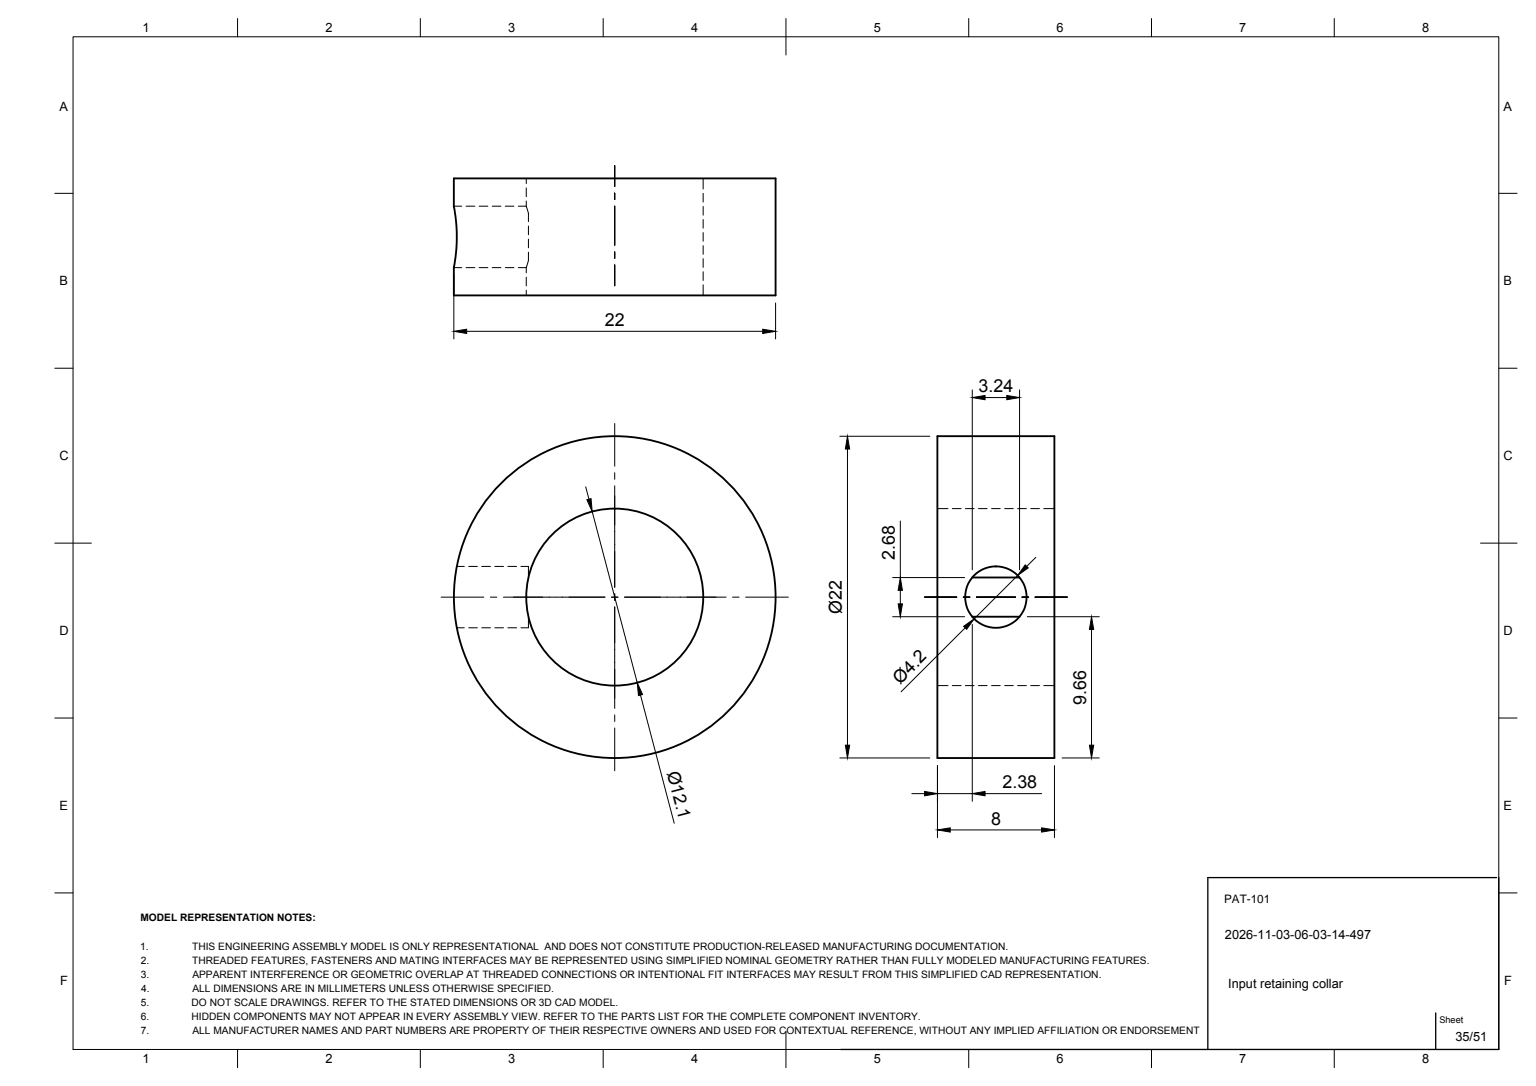
ISO-10303-21;
HEADER;
/* Generated by software containing ST-Developer
 * from STEP Tools, Inc. (www.steptools.com) 
 */

FILE_DESCRIPTION(
/* description */ ('Spur gear reduction stage 2-1 on bearing plates'),
/* implementation_level */ '2;1');

FILE_NAME(
/* name */ 'Input retaining collar.step',
/* time_stamp */ '2026-10-28T03:22:07-07:00',
/* author */ (''),
/* organization */ (''),
/* preprocessor_version */ 'ST-DEVELOPER v20.2',
/* originating_system */ 'Autodesk Translation Framework v15.17.0.0',
/* authorisation */ '');

FILE_SCHEMA (('AUTOMOTIVE_DESIGN { 1 0 10303 214 3 1 1 }'));
ENDSEC;

DATA;
#10=MECHANICAL_DESIGN_GEOMETRIC_PRESENTATION_REPRESENTATION('',(#989),#53909);
#699=B_SPLINE_CURVE_WITH_KNOTS('',3,(#17992,#17993,#17994,#17995,#17996,
#17997,#17998,#17999,#18000,#18001),.UNSPECIFIED.,.F.,.F.,(4,2,2,2,4),(0.818088904349169,
0.878131747417165,0.957937926194036,1.03774410497091,1.0977869480389),
 .UNSPECIFIED.);
#700=B_SPLINE_CURVE_WITH_KNOTS('',3,(#18007,#18008,#18009,#18010,#18011,
#18012,#18013,#18014,#18015,#18016,#18017,#18018,#18019,#18020,#18021,#18022,
#18023,#18024),.UNSPECIFIED.,.F.,.F.,(4,2,2,2,2,2,2,2,4),(0.,0.0793157643915219,
0.158631528783044,0.23794361593365,0.317255703084255,0.396567790234861,
0.475879877385467,0.555195641776989,0.634511406168511),.UNSPECIFIED.);
#701=B_SPLINE_CURVE_WITH_KNOTS('',3,(#18025,#18026,#18027,#18028,#18029,
#18030,#18031,#18032,#18033,#18034,#18035,#18036,#18037,#18038,#18039,#18040,
#18041,#18042),.UNSPECIFIED.,.F.,.F.,(4,2,2,2,2,2,2,2,4),(0.634511406168511,
0.713827170560033,0.793142934951554,0.87245502210216,0.951767109252766,
1.03107919640337,1.11039128355398,1.1897070479455,1.26902281233702),
 .UNSPECIFIED.);
#702=B_SPLINE_CURVE_WITH_KNOTS('',3,(#18045,#18046,#18047,#18048,#18049,
#18050,#18051,#18052,#18053,#18054),.UNSPECIFIED.,.F.,.F.,(4,2,2,2,4),(0.179463620219812,
0.239506463287808,0.319312642064679,0.399118820841549,0.459161663909545),
 .UNSPECIFIED.);
#888=SHAPE_REPRESENTATION_RELATIONSHIP('SRR','None',#54118,#931);
#931=ADVANCED_BREP_SHAPE_REPRESENTATION('',(#1044),#53892);
#989=STYLED_ITEM('',(#54383),#1044);
#1044=MANIFOLD_SOLID_BREP('Body1',#11316);
#1202=FACE_BOUND('',#2593,.T.);
#1203=FACE_BOUND('',#2595,.T.);
#1204=FACE_BOUND('',#2597,.T.);
#1205=FACE_BOUND('',#2599,.T.);
#1369=PLANE('',#12513);
#1370=PLANE('',#12518);
#1371=PLANE('',#12525);
#1372=PLANE('',#12526);
#1799=FACE_OUTER_BOUND('',#2589,.T.);
#1800=FACE_OUTER_BOUND('',#2590,.T.);
#1801=FACE_OUTER_BOUND('',#2591,.T.);
#1802=FACE_OUTER_BOUND('',#2592,.T.);
#1803=FACE_OUTER_BOUND('',#2594,.T.);
#1804=FACE_OUTER_BOUND('',#2596,.T.);
#1805=FACE_OUTER_BOUND('',#2598,.T.);
#2589=EDGE_LOOP('',(#8536,#8537));
#2590=EDGE_LOOP('',(#8538,#8539,#8540,#8541,#8542,#8543,#8544,#8545,#8546));
#2591=EDGE_LOOP('',(#8547,#8548,#8549));
#2592=EDGE_LOOP('',(#8550,#8551,#8552,#8553));
#2593=EDGE_LOOP('',(#8554,#8555,#8556,#8557));
#2594=EDGE_LOOP('',(#8558,#8559,#8560,#8561));
#2595=EDGE_LOOP('',(#8562,#8563));
#2596=EDGE_LOOP('',(#8564));
#2597=EDGE_LOOP('',(#8565));
#2598=EDGE_LOOP('',(#8566));
#2599=EDGE_LOOP('',(#8567));
#3208=LINE('',#17988,#3849);
#3209=LINE('',#18005,#3850);
#3210=LINE('',#18056,#3851);
#3211=LINE('',#18061,#3852);
#3212=LINE('',#18067,#3853);
#3849=VECTOR('',#14629,1.);
#3850=VECTOR('',#14636,0.21);
#3851=VECTOR('',#14641,1.);
#3852=VECTOR('',#14646,0.605);
#3853=VECTOR('',#14653,1.1);
#4588=CIRCLE('',#12514,0.21);
#4589=CIRCLE('',#12516,0.21);
#4590=CIRCLE('',#12517,0.21);
#4591=CIRCLE('',#12520,0.605);
#4592=CIRCLE('',#12521,0.605);
#4593=CIRCLE('',#12523,1.1);
#4594=CIRCLE('',#12524,1.1);
#5192=VERTEX_POINT('',#17986);
#5193=VERTEX_POINT('',#17987);
#5194=VERTEX_POINT('',#17991);
#5195=VERTEX_POINT('',#18002);
#5196=VERTEX_POINT('',#18004);
#5197=VERTEX_POINT('',#18006);
#5198=VERTEX_POINT('',#18043);
#5199=VERTEX_POINT('',#18058);
#5200=VERTEX_POINT('',#18060);
#5201=VERTEX_POINT('',#18064);
#5202=VERTEX_POINT('',#18066);
#6410=EDGE_CURVE('',#5192,#5193,#3208,.T.);
#6411=EDGE_CURVE('',#5192,#5193,#4588,.T.);
#6412=EDGE_CURVE('',#5194,#5192,#699,.T.);
#6413=EDGE_CURVE('',#5195,#5194,#4589,.T.);
#6414=EDGE_CURVE('',#5195,#5196,#3209,.T.);
#6415=EDGE_CURVE('',#5197,#5196,#700,.T.);
#6416=EDGE_CURVE('',#5196,#5197,#701,.T.);
#6417=EDGE_CURVE('',#5198,#5195,#4590,.T.);
#6418=EDGE_CURVE('',#5193,#5198,#702,.T.);
#6419=EDGE_CURVE('',#5198,#5194,#3210,.T.);
#6420=EDGE_CURVE('',#5199,#5199,#4591,.T.);
#6421=EDGE_CURVE('',#5199,#5200,#3211,.T.);
#6422=EDGE_CURVE('',#5200,#5200,#4592,.T.);
#6423=EDGE_CURVE('',#5201,#5201,#4593,.T.);
#6424=EDGE_CURVE('',#5201,#5202,#3212,.T.);
#6425=EDGE_CURVE('',#5202,#5202,#4594,.T.);
#8536=ORIENTED_EDGE('',*,*,#6410,.F.);
#8537=ORIENTED_EDGE('',*,*,#6411,.T.);
#8538=ORIENTED_EDGE('',*,*,#6412,.F.);
#8539=ORIENTED_EDGE('',*,*,#6413,.F.);
#8540=ORIENTED_EDGE('',*,*,#6414,.T.);
#8541=ORIENTED_EDGE('',*,*,#6415,.F.);
#8542=ORIENTED_EDGE('',*,*,#6416,.F.);
#8543=ORIENTED_EDGE('',*,*,#6414,.F.);
#8544=ORIENTED_EDGE('',*,*,#6417,.F.);
#8545=ORIENTED_EDGE('',*,*,#6418,.F.);
#8546=ORIENTED_EDGE('',*,*,#6411,.F.);
#8547=ORIENTED_EDGE('',*,*,#6419,.F.);
#8548=ORIENTED_EDGE('',*,*,#6417,.T.);
#8549=ORIENTED_EDGE('',*,*,#6413,.T.);
#8550=ORIENTED_EDGE('',*,*,#6420,.F.);
#8551=ORIENTED_EDGE('',*,*,#6421,.T.);
#8552=ORIENTED_EDGE('',*,*,#6422,.T.);
#8553=ORIENTED_EDGE('',*,*,#6421,.F.);
#8554=ORIENTED_EDGE('',*,*,#6418,.T.);
#8555=ORIENTED_EDGE('',*,*,#6419,.T.);
#8556=ORIENTED_EDGE('',*,*,#6412,.T.);
#8557=ORIENTED_EDGE('',*,*,#6410,.T.);
#8558=ORIENTED_EDGE('',*,*,#6423,.F.);
#8559=ORIENTED_EDGE('',*,*,#6424,.T.);
#8560=ORIENTED_EDGE('',*,*,#6425,.T.);
#8561=ORIENTED_EDGE('',*,*,#6424,.F.);
#8562=ORIENTED_EDGE('',*,*,#6415,.T.);
#8563=ORIENTED_EDGE('',*,*,#6416,.T.);
#8564=ORIENTED_EDGE('',*,*,#6423,.T.);
#8565=ORIENTED_EDGE('',*,*,#6420,.T.);
#8566=ORIENTED_EDGE('',*,*,#6425,.F.);
#8567=ORIENTED_EDGE('',*,*,#6422,.F.);
#10531=CYLINDRICAL_SURFACE('',#12515,0.21);
#10532=CYLINDRICAL_SURFACE('',#12519,0.605);
#10533=CYLINDRICAL_SURFACE('',#12522,1.1);
#10919=ADVANCED_FACE('',(#1799),#1369,.T.);
#10920=ADVANCED_FACE('',(#1800),#10531,.F.);
#10921=ADVANCED_FACE('',(#1801),#1370,.T.);
#10922=ADVANCED_FACE('',(#1802,#1202),#10532,.F.);
#10923=ADVANCED_FACE('',(#1803,#1203),#10533,.T.);
#10924=ADVANCED_FACE('',(#1804,#1204),#1371,.T.);
#10925=ADVANCED_FACE('',(#1805,#1205),#1372,.F.);
#11316=CLOSED_SHELL('',(#10919,#10920,#10921,#10922,#10923,#10924,#10925));
#12512=AXIS2_PLACEMENT_3D('',#17984,#14625,#14626);
#12513=AXIS2_PLACEMENT_3D('',#17985,#14627,#14628);
#12514=AXIS2_PLACEMENT_3D('',#17989,#14630,#14631);
#12515=AXIS2_PLACEMENT_3D('',#17990,#14632,#14633);
#12516=AXIS2_PLACEMENT_3D('',#18003,#14634,#14635);
#12517=AXIS2_PLACEMENT_3D('',#18044,#14637,#14638);
#12518=AXIS2_PLACEMENT_3D('',#18055,#14639,#14640);
#12519=AXIS2_PLACEMENT_3D('',#18057,#14642,#14643);
#12520=AXIS2_PLACEMENT_3D('',#18059,#14644,#14645);
#12521=AXIS2_PLACEMENT_3D('',#18062,#14647,#14648);
#12522=AXIS2_PLACEMENT_3D('',#18063,#14649,#14650);
#12523=AXIS2_PLACEMENT_3D('',#18065,#14651,#14652);
#12524=AXIS2_PLACEMENT_3D('',#18068,#14654,#14655);
#12525=AXIS2_PLACEMENT_3D('',#18069,#14656,#14657);
#12526=AXIS2_PLACEMENT_3D('',#18070,#14658,#14659);
#14625=DIRECTION('axis',(0.,0.,1.));
#14626=DIRECTION('refdir',(1.,0.,0.));
#14627=DIRECTION('center_axis',(0.,0.,1.));
#14628=DIRECTION('ref_axis',(1.,0.,0.));
#14629=DIRECTION('',(0.,1.,0.));
#14630=DIRECTION('center_axis',(0.,0.,1.));
#14631=DIRECTION('ref_axis',(1.,0.,0.));
#14632=DIRECTION('center_axis',(0.,0.,1.));
#14633=DIRECTION('ref_axis',(1.,0.,0.));
#14634=DIRECTION('center_axis',(0.,0.,1.));
#14635=DIRECTION('ref_axis',(1.,0.,0.));
#14636=DIRECTION('',(0.,0.,1.));
#14637=DIRECTION('center_axis',(0.,0.,1.));
#14638=DIRECTION('ref_axis',(1.,0.,0.));
#14639=DIRECTION('center_axis',(0.,0.,1.));
#14640=DIRECTION('ref_axis',(1.,0.,0.));
#14641=DIRECTION('',(0.,-1.,0.));
#14642=DIRECTION('center_axis',(0.,1.,0.));
#14643=DIRECTION('ref_axis',(1.,0.,0.));
#14644=DIRECTION('center_axis',(0.,-1.,0.));
#14645=DIRECTION('ref_axis',(1.,0.,0.));
#14646=DIRECTION('',(0.,-1.,0.));
#14647=DIRECTION('center_axis',(0.,-1.,0.));
#14648=DIRECTION('ref_axis',(1.,0.,0.));
#14649=DIRECTION('center_axis',(0.,1.,0.));
#14650=DIRECTION('ref_axis',(1.,0.,0.));
#14651=DIRECTION('center_axis',(0.,1.,0.));
#14652=DIRECTION('ref_axis',(1.,0.,0.));
#14653=DIRECTION('',(0.,-1.,0.));
#14654=DIRECTION('center_axis',(0.,1.,0.));
#14655=DIRECTION('ref_axis',(1.,0.,0.));
#14656=DIRECTION('center_axis',(0.,1.,0.));
#14657=DIRECTION('ref_axis',(1.,0.,0.));
#14658=DIRECTION('center_axis',(0.,1.,0.));
#14659=DIRECTION('ref_axis',(1.,0.,0.));
#17984=CARTESIAN_POINT('',(0.,0.,0.));
#17985=CARTESIAN_POINT('Origin',(0.,-5.1,0.59));
#17986=CARTESIAN_POINT('',(0.133884278389959,-5.26178689687363,0.59));
#17987=CARTESIAN_POINT('',(0.133884278389959,-4.93821310312637,0.59));
#17988=CARTESIAN_POINT('',(0.133884278389959,-5.5,0.59));
#17989=CARTESIAN_POINT('Origin',(0.,-5.1,0.59));
#17990=CARTESIAN_POINT('Origin',(0.,-5.1,0.59));
#17991=CARTESIAN_POINT('',(-0.133884278389959,-5.26178689687363,0.59));
#17992=CARTESIAN_POINT('Ctrl Pts',(-0.133884278389959,-5.26178689687363,
0.59));
#17993=CARTESIAN_POINT('Ctrl Pts',(-0.118254395260804,-5.27472116821763,
0.59354677224418));
#17994=CARTESIAN_POINT('Ctrl Pts',(-0.1001097876823,-5.28579931658744,0.596982247899573));
#17995=CARTESIAN_POINT('Ctrl Pts',(-0.0548298721325195,-5.30463856105443,
0.603074162899704));
#17996=CARTESIAN_POINT('Ctrl Pts',(-0.0266020595922903,-5.31,0.605));
#17997=CARTESIAN_POINT('Ctrl Pts',(0.0266020595922903,-5.31,0.605));
#17998=CARTESIAN_POINT('Ctrl Pts',(0.0548298721325197,-5.30463856105443,
0.603074162899704));
#17999=CARTESIAN_POINT('Ctrl Pts',(0.100109787682301,-5.28579931658744,
0.596982247899573));
#18000=CARTESIAN_POINT('Ctrl Pts',(0.118254395260804,-5.27472116821763,
0.59354677224418));
#18001=CARTESIAN_POINT('Ctrl Pts',(0.133884278389959,-5.26178689687363,
0.59));
#18002=CARTESIAN_POINT('',(-0.21,-5.1,0.59));
#18003=CARTESIAN_POINT('Origin',(0.,-5.1,0.59));
#18004=CARTESIAN_POINT('',(-0.21,-5.1,1.07976849370594));
#18005=CARTESIAN_POINT('',(-0.21,-5.1,0.59));
#18006=CARTESIAN_POINT('',(0.21,-5.1,1.07976849370594));
#18007=CARTESIAN_POINT('Ctrl Pts',(0.21,-5.1,1.07976849370594));
#18008=CARTESIAN_POINT('Ctrl Pts',(0.21,-5.12643858813051,1.07976849370594));
#18009=CARTESIAN_POINT('Ctrl Pts',(0.204702922670977,-5.15459378125493,
1.08084015664674));
#18010=CARTESIAN_POINT('Ctrl Pts',(0.183251796806355,-5.20631344554134,
1.08468313707126));
#18011=CARTESIAN_POINT('Ctrl Pts',(0.167101177357215,-5.22988367074114,
1.08739593054622));
#18012=CARTESIAN_POINT('Ctrl Pts',(0.129884533480965,-5.26710031461738,
1.09246633289124));
#18013=CARTESIAN_POINT('Ctrl Pts',(0.106313940757289,-5.28325161016341,
1.09515738895358));
#18014=CARTESIAN_POINT('Ctrl Pts',(0.0545930033295209,-5.30470322656974,
1.09895039220591));
#18015=CARTESIAN_POINT('Ctrl Pts',(0.0264373623835353,-5.31,1.1));
#18016=CARTESIAN_POINT('Ctrl Pts',(-0.0264373623835352,-5.31,1.1));
#18017=CARTESIAN_POINT('Ctrl Pts',(-0.0545930033295208,-5.30470322656974,
1.09895039220591));
#18018=CARTESIAN_POINT('Ctrl Pts',(-0.106313940757289,-5.28325161016341,
1.09515738895358));
#18019=CARTESIAN_POINT('Ctrl Pts',(-0.129884533480965,-5.26710031461738,
1.09246633289124));
#18020=CARTESIAN_POINT('Ctrl Pts',(-0.167101177357215,-5.22988367074114,
1.08739593054622));
#18021=CARTESIAN_POINT('Ctrl Pts',(-0.183251796806354,-5.20631344554134,
1.08468313707126));
#18022=CARTESIAN_POINT('Ctrl Pts',(-0.204702922670976,-5.15459378125493,
1.08084015664674));
#18023=CARTESIAN_POINT('Ctrl Pts',(-0.21,-5.12643858813051,1.07976849370594));
#18024=CARTESIAN_POINT('Ctrl Pts',(-0.21,-5.1,1.07976849370594));
#18025=CARTESIAN_POINT('Ctrl Pts',(-0.21,-5.1,1.07976849370594));
#18026=CARTESIAN_POINT('Ctrl Pts',(-0.21,-5.07356141186949,1.07976849370594));
#18027=CARTESIAN_POINT('Ctrl Pts',(-0.204702922670977,-5.04540621874507,
1.08084015664674));
#18028=CARTESIAN_POINT('Ctrl Pts',(-0.183251796806355,-4.99368655445866,
1.08468313707126));
#18029=CARTESIAN_POINT('Ctrl Pts',(-0.167101177357215,-4.97011632925886,
1.08739593054622));
#18030=CARTESIAN_POINT('Ctrl Pts',(-0.129884533480965,-4.93289968538261,
1.09246633289124));
#18031=CARTESIAN_POINT('Ctrl Pts',(-0.106313940757289,-4.91674838983659,
1.09515738895358));
#18032=CARTESIAN_POINT('Ctrl Pts',(-0.0545930033295209,-4.89529677343026,
1.09895039220591));
#18033=CARTESIAN_POINT('Ctrl Pts',(-0.0264373623835353,-4.89,1.1));
#18034=CARTESIAN_POINT('Ctrl Pts',(0.0264373623835353,-4.89,1.1));
#18035=CARTESIAN_POINT('Ctrl Pts',(0.0545930033295197,-4.89529677343026,
1.09895039220591));
#18036=CARTESIAN_POINT('Ctrl Pts',(0.106313940757288,-4.91674838983659,
1.09515738895358));
#18037=CARTESIAN_POINT('Ctrl Pts',(0.129884533480965,-4.93289968538261,
1.09246633289124));
#18038=CARTESIAN_POINT('Ctrl Pts',(0.167101177357214,-4.97011632925886,
1.08739593054622));
#18039=CARTESIAN_POINT('Ctrl Pts',(0.183251796806355,-4.99368655445866,
1.08468313707126));
#18040=CARTESIAN_POINT('Ctrl Pts',(0.204702922670977,-5.04540621874507,
1.08084015664674));
#18041=CARTESIAN_POINT('Ctrl Pts',(0.21,-5.07356141186949,1.07976849370594));
#18042=CARTESIAN_POINT('Ctrl Pts',(0.21,-5.1,1.07976849370594));
#18043=CARTESIAN_POINT('',(-0.133884278389959,-4.93821310312637,0.59));
#18044=CARTESIAN_POINT('Origin',(0.,-5.1,0.59));
#18045=CARTESIAN_POINT('Ctrl Pts',(0.133884278389959,-4.93821310312637,
0.59));
#18046=CARTESIAN_POINT('Ctrl Pts',(0.118254395260804,-4.92527883178237,
0.59354677224418));
#18047=CARTESIAN_POINT('Ctrl Pts',(0.1001097876823,-4.91420068341256,0.596982247899573));
#18048=CARTESIAN_POINT('Ctrl Pts',(0.0548298721325194,-4.89536143894557,
0.603074162899704));
#18049=CARTESIAN_POINT('Ctrl Pts',(0.0266020595922903,-4.89,0.605));
#18050=CARTESIAN_POINT('Ctrl Pts',(-0.0266020595922903,-4.89,0.605));
#18051=CARTESIAN_POINT('Ctrl Pts',(-0.0548298721325194,-4.89536143894557,
0.603074162899704));
#18052=CARTESIAN_POINT('Ctrl Pts',(-0.1001097876823,-4.91420068341256,0.596982247899573));
#18053=CARTESIAN_POINT('Ctrl Pts',(-0.118254395260804,-4.92527883178237,
0.59354677224418));
#18054=CARTESIAN_POINT('Ctrl Pts',(-0.133884278389959,-4.93821310312636,
0.59));
#18055=CARTESIAN_POINT('Origin',(0.,-5.1,0.59));
#18056=CARTESIAN_POINT('',(-0.133884278389959,-5.5,0.59));
#18057=CARTESIAN_POINT('Origin',(0.,-5.5,0.));
#18058=CARTESIAN_POINT('',(-0.605,-4.7,7.40911313484149E-17));
#18059=CARTESIAN_POINT('Origin',(0.,-4.7,0.));
#18060=CARTESIAN_POINT('',(-0.605,-5.5,7.40911313484149E-17));
#18061=CARTESIAN_POINT('',(-0.605,-5.5,7.40911313484149E-17));
#18062=CARTESIAN_POINT('Origin',(0.,-5.5,0.));
#18063=CARTESIAN_POINT('Origin',(0.,-5.5,0.));
#18064=CARTESIAN_POINT('',(-1.1,-4.7,1.34711147906209E-16));
#18065=CARTESIAN_POINT('Origin',(0.,-4.7,0.));
#18066=CARTESIAN_POINT('',(-1.1,-5.5,1.34711147906209E-16));
#18067=CARTESIAN_POINT('',(-1.1,-5.5,1.34711147906209E-16));
#18068=CARTESIAN_POINT('Origin',(0.,-5.5,0.));
#18069=CARTESIAN_POINT('Origin',(0.,-4.7,0.));
#18070=CARTESIAN_POINT('Origin',(0.,-5.5,0.));
#53842=UNCERTAINTY_MEASURE_WITH_UNIT(LENGTH_MEASURE(0.001),#53910,
'DISTANCE_ACCURACY_VALUE',
'Maximum model space distance between geometric entities at asserted c
onnectivities');
#53859=UNCERTAINTY_MEASURE_WITH_UNIT(LENGTH_MEASURE(0.001),#53910,
'DISTANCE_ACCURACY_VALUE',
'Maximum model space distance between geometric entities at asserted c
onnectivities');
#53892=(
GEOMETRIC_REPRESENTATION_CONTEXT(3)
GLOBAL_UNCERTAINTY_ASSIGNED_CONTEXT((#53842))
GLOBAL_UNIT_ASSIGNED_CONTEXT((#53910,#53912,#53913))
REPRESENTATION_CONTEXT('','3D')
);
#53909=(
GEOMETRIC_REPRESENTATION_CONTEXT(3)
GLOBAL_UNCERTAINTY_ASSIGNED_CONTEXT((#53859))
GLOBAL_UNIT_ASSIGNED_CONTEXT((#53910,#53912,#53913))
REPRESENTATION_CONTEXT('','3D')
);
#53910=(
LENGTH_UNIT()
NAMED_UNIT(*)
SI_UNIT(.CENTI.,.METRE.)
);
#53912=(
NAMED_UNIT(*)
PLANE_ANGLE_UNIT()
SI_UNIT($,.RADIAN.)
);
#53913=(
NAMED_UNIT(*)
SI_UNIT($,.STERADIAN.)
SOLID_ANGLE_UNIT()
);
#53946=SHAPE_DEFINITION_REPRESENTATION(#54044,#54118);
#54044=PRODUCT_DEFINITION_SHAPE('',$,#54168);
#54118=SHAPE_REPRESENTATION('',(#12512),#53892);
#54135=PRODUCT_DEFINITION_CONTEXT('part definition',#54284,'design');
#54168=PRODUCT_DEFINITION('Input retaining collar',
'Input retaining collar',#54217,#54135);
#54217=PRODUCT_DEFINITION_FORMATION('',$,#54318);
#54284=APPLICATION_CONTEXT(
'Core Data for Automotive Mechanical Design Process');
#54285=PRODUCT_CONTEXT('part definition',#54284,'mechanical');
#54318=PRODUCT('Input retaining collar','Input retaining collar',
'Input retaining collar',(#54285));
#54377=COLOUR_RGB('Light Blue',0.38,0.62,0.78);
#54378=FILL_AREA_STYLE_COLOUR('',#54377);
#54379=FILL_AREA_STYLE('',(#54378));
#54380=SURFACE_STYLE_FILL_AREA(#54379);
#54381=SURFACE_SIDE_STYLE('',(#54380));
#54382=SURFACE_STYLE_USAGE(.BOTH.,#54381);
#54383=PRESENTATION_STYLE_ASSIGNMENT((#54382));
ENDSEC;
END-ISO-10303-21;
